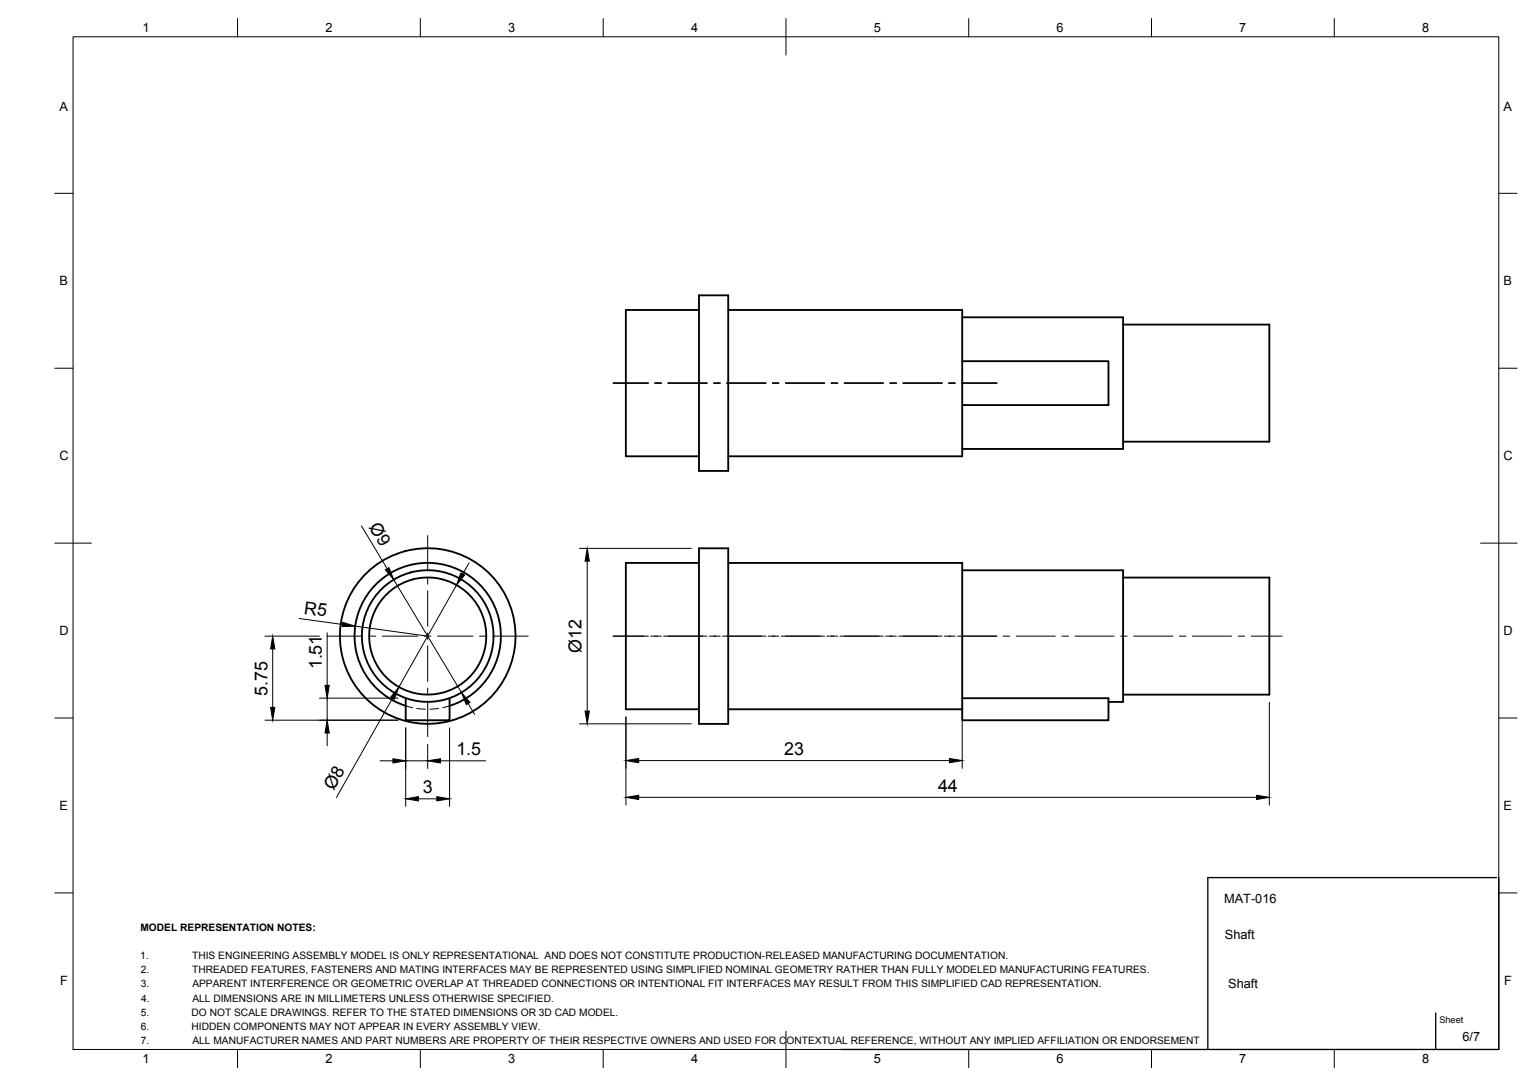
ISO-10303-21;
HEADER;
/* Generated by software containing ST-Developer
 * from STEP Tools, Inc. (www.steptools.com) 
 */

FILE_DESCRIPTION(
/* description */ ('STEP AP214'),
/* implementation_level */ '2;1');

FILE_NAME(
/* name */ 'Shaft.step',
/* time_stamp */ '2026-11-14T06:10:26-08:00',
/* author */ (''),
/* organization */ (''),
/* preprocessor_version */ 'ST-DEVELOPER v20.2',
/* originating_system */ 'Autodesk Translation Framework v15.17.0.0',
/* authorisation */ '');

FILE_SCHEMA (('AUTOMOTIVE_DESIGN { 1 0 10303 214 3 1 1 }'));
ENDSEC;

DATA;
#10=MECHANICAL_DESIGN_GEOMETRIC_PRESENTATION_REPRESENTATION('',(#165),#10413);
#149=SHAPE_REPRESENTATION_RELATIONSHIP('SRR','None',#10454,#157);
#157=ADVANCED_BREP_SHAPE_REPRESENTATION('',(#173),#10406);
#165=STYLED_ITEM('',(#10502),#173);
#173=MANIFOLD_SOLID_BREP('Body1',#5300);
#196=FACE_BOUND('',#606,.T.);
#197=FACE_BOUND('',#608,.T.);
#198=FACE_BOUND('',#611,.T.);
#229=PLANE('',#5455);
#230=PLANE('',#5456);
#231=PLANE('',#5457);
#232=PLANE('',#5458);
#233=PLANE('',#5459);
#234=PLANE('',#5460);
#235=PLANE('',#5461);
#236=PLANE('',#5462);
#237=PLANE('',#5463);
#238=PLANE('',#5464);
#239=PLANE('',#5465);
#294=FACE_OUTER_BOUND('',#600,.T.);
#295=FACE_OUTER_BOUND('',#601,.T.);
#296=FACE_OUTER_BOUND('',#602,.T.);
#297=FACE_OUTER_BOUND('',#603,.T.);
#298=FACE_OUTER_BOUND('',#604,.T.);
#299=FACE_OUTER_BOUND('',#605,.T.);
#300=FACE_OUTER_BOUND('',#607,.T.);
#301=FACE_OUTER_BOUND('',#609,.T.);
#302=FACE_OUTER_BOUND('',#610,.T.);
#303=FACE_OUTER_BOUND('',#612,.T.);
#304=FACE_OUTER_BOUND('',#613,.T.);
#305=FACE_OUTER_BOUND('',#614,.T.);
#306=FACE_OUTER_BOUND('',#615,.T.);
#307=FACE_OUTER_BOUND('',#616,.T.);
#308=FACE_OUTER_BOUND('',#617,.T.);
#309=FACE_OUTER_BOUND('',#618,.T.);
#600=EDGE_LOOP('',(#3312,#3313,#3314,#3315));
#601=EDGE_LOOP('',(#3316,#3317,#3318,#3319,#3320,#3321,#3322,#3323));
#602=EDGE_LOOP('',(#3324,#3325,#3326,#3327,#3328,#3329));
#603=EDGE_LOOP('',(#3330,#3331,#3332,#3333));
#604=EDGE_LOOP('',(#3334,#3335,#3336,#3337));
#605=EDGE_LOOP('',(#3338));
#606=EDGE_LOOP('',(#3339));
#607=EDGE_LOOP('',(#3340));
#608=EDGE_LOOP('',(#3341));
#609=EDGE_LOOP('',(#3342));
#610=EDGE_LOOP('',(#3343));
#611=EDGE_LOOP('',(#3344));
#612=EDGE_LOOP('',(#3345,#3346,#3347,#3348,#3349,#3350));
#613=EDGE_LOOP('',(#3351,#3352,#3353,#3354));
#614=EDGE_LOOP('',(#3355,#3356,#3357,#3358,#3359));
#615=EDGE_LOOP('',(#3360,#3361,#3362,#3363));
#616=EDGE_LOOP('',(#3364,#3365,#3366,#3367,#3368));
#617=EDGE_LOOP('',(#3369,#3370,#3371,#3372));
#618=EDGE_LOOP('',(#3373));
#921=LINE('',#8050,#1212);
#922=LINE('',#8057,#1213);
#923=LINE('',#8061,#1214);
#924=LINE('',#8065,#1215);
#925=LINE('',#8070,#1216);
#926=LINE('',#8080,#1217);
#927=LINE('',#8086,#1218);
#928=LINE('',#8093,#1219);
#929=LINE('',#8094,#1220);
#930=LINE('',#8097,#1221);
#931=LINE('',#8099,#1222);
#932=LINE('',#8100,#1223);
#933=LINE('',#8103,#1224);
#934=LINE('',#8104,#1225);
#935=LINE('',#8107,#1226);
#936=LINE('',#8108,#1227);
#937=LINE('',#8110,#1228);
#1212=VECTOR('',#6261,4.);
#1213=VECTOR('',#6268,1000.);
#1214=VECTOR('',#6271,4.5);
#1215=VECTOR('',#6276,1000.);
#1216=VECTOR('',#6281,5.);
#1217=VECTOR('',#6292,6.);
#1218=VECTOR('',#6299,5.);
#1219=VECTOR('',#6312,1000.);
#1220=VECTOR('',#6313,1000.);
#1221=VECTOR('',#6316,1000.);
#1222=VECTOR('',#6317,1000.);
#1223=VECTOR('',#6318,1000.);
#1224=VECTOR('',#6321,1000.);
#1225=VECTOR('',#6322,1000.);
#1226=VECTOR('',#6325,1000.);
#1227=VECTOR('',#6326,1000.);
#1228=VECTOR('',#6329,1000.);
#1494=CIRCLE('',#5437,4.);
#1495=CIRCLE('',#5438,4.);
#1496=CIRCLE('',#5440,4.5);
#1497=CIRCLE('',#5441,4.5);
#1498=CIRCLE('',#5442,4.5);
#1499=CIRCLE('',#5443,4.5);
#1500=CIRCLE('',#5445,5.);
#1501=CIRCLE('',#5446,5.);
#1502=CIRCLE('',#5447,5.);
#1503=CIRCLE('',#5448,5.);
#1504=CIRCLE('',#5450,6.);
#1505=CIRCLE('',#5451,6.);
#1506=CIRCLE('',#5453,5.);
#1507=CIRCLE('',#5454,5.);
#1947=VERTEX_POINT('',#8047);
#1948=VERTEX_POINT('',#8049);
#1949=VERTEX_POINT('',#8053);
#1950=VERTEX_POINT('',#8054);
#1951=VERTEX_POINT('',#8056);
#1952=VERTEX_POINT('',#8058);
#1953=VERTEX_POINT('',#8060);
#1954=VERTEX_POINT('',#8063);
#1955=VERTEX_POINT('',#8067);
#1956=VERTEX_POINT('',#8069);
#1957=VERTEX_POINT('',#8071);
#1958=VERTEX_POINT('',#8073);
#1959=VERTEX_POINT('',#8077);
#1960=VERTEX_POINT('',#8079);
#1961=VERTEX_POINT('',#8083);
#1962=VERTEX_POINT('',#8085);
#1963=VERTEX_POINT('',#8096);
#1964=VERTEX_POINT('',#8098);
#1965=VERTEX_POINT('',#8102);
#1966=VERTEX_POINT('',#8106);
#2481=EDGE_CURVE('',#1947,#1947,#1494,.T.);
#2482=EDGE_CURVE('',#1947,#1948,#921,.T.);
#2483=EDGE_CURVE('',#1948,#1948,#1495,.T.);
#2484=EDGE_CURVE('',#1949,#1950,#1496,.T.);
#2485=EDGE_CURVE('',#1950,#1951,#922,.T.);
#2486=EDGE_CURVE('',#1951,#1952,#1497,.T.);
#2487=EDGE_CURVE('',#1952,#1953,#923,.T.);
#2488=EDGE_CURVE('',#1953,#1953,#1498,.T.);
#2489=EDGE_CURVE('',#1952,#1954,#1499,.T.);
#2490=EDGE_CURVE('',#1949,#1954,#924,.T.);
#2491=EDGE_CURVE('',#1955,#1955,#1500,.T.);
#2492=EDGE_CURVE('',#1955,#1956,#925,.T.);
#2493=EDGE_CURVE('',#1957,#1956,#1501,.T.);
#2494=EDGE_CURVE('',#1958,#1957,#1502,.T.);
#2495=EDGE_CURVE('',#1956,#1958,#1503,.T.);
#2496=EDGE_CURVE('',#1959,#1959,#1504,.T.);
#2497=EDGE_CURVE('',#1959,#1960,#926,.T.);
#2498=EDGE_CURVE('',#1960,#1960,#1505,.T.);
#2499=EDGE_CURVE('',#1961,#1961,#1506,.T.);
#2500=EDGE_CURVE('',#1961,#1962,#927,.T.);
#2501=EDGE_CURVE('',#1962,#1962,#1507,.T.);
#2502=EDGE_CURVE('',#1954,#1958,#928,.T.);
#2503=EDGE_CURVE('',#1957,#1951,#929,.T.);
#2504=EDGE_CURVE('',#1958,#1963,#930,.T.);
#2505=EDGE_CURVE('',#1964,#1957,#931,.T.);
#2506=EDGE_CURVE('',#1963,#1964,#932,.T.);
#2507=EDGE_CURVE('',#1965,#1963,#933,.T.);
#2508=EDGE_CURVE('',#1949,#1965,#934,.T.);
#2509=EDGE_CURVE('',#1966,#1964,#935,.T.);
#2510=EDGE_CURVE('',#1965,#1966,#936,.T.);
#2511=EDGE_CURVE('',#1966,#1950,#937,.T.);
#3312=ORIENTED_EDGE('',*,*,#2481,.T.);
#3313=ORIENTED_EDGE('',*,*,#2482,.T.);
#3314=ORIENTED_EDGE('',*,*,#2483,.F.);
#3315=ORIENTED_EDGE('',*,*,#2482,.F.);
#3316=ORIENTED_EDGE('',*,*,#2484,.T.);
#3317=ORIENTED_EDGE('',*,*,#2485,.T.);
#3318=ORIENTED_EDGE('',*,*,#2486,.T.);
#3319=ORIENTED_EDGE('',*,*,#2487,.T.);
#3320=ORIENTED_EDGE('',*,*,#2488,.F.);
#3321=ORIENTED_EDGE('',*,*,#2487,.F.);
#3322=ORIENTED_EDGE('',*,*,#2489,.T.);
#3323=ORIENTED_EDGE('',*,*,#2490,.F.);
#3324=ORIENTED_EDGE('',*,*,#2491,.T.);
#3325=ORIENTED_EDGE('',*,*,#2492,.T.);
#3326=ORIENTED_EDGE('',*,*,#2493,.F.);
#3327=ORIENTED_EDGE('',*,*,#2494,.F.);
#3328=ORIENTED_EDGE('',*,*,#2495,.F.);
#3329=ORIENTED_EDGE('',*,*,#2492,.F.);
#3330=ORIENTED_EDGE('',*,*,#2496,.T.);
#3331=ORIENTED_EDGE('',*,*,#2497,.T.);
#3332=ORIENTED_EDGE('',*,*,#2498,.F.);
#3333=ORIENTED_EDGE('',*,*,#2497,.F.);
#3334=ORIENTED_EDGE('',*,*,#2499,.T.);
#3335=ORIENTED_EDGE('',*,*,#2500,.T.);
#3336=ORIENTED_EDGE('',*,*,#2501,.F.);
#3337=ORIENTED_EDGE('',*,*,#2500,.F.);
#3338=ORIENTED_EDGE('',*,*,#2488,.T.);
#3339=ORIENTED_EDGE('',*,*,#2481,.F.);
#3340=ORIENTED_EDGE('',*,*,#2498,.T.);
#3341=ORIENTED_EDGE('',*,*,#2491,.F.);
#3342=ORIENTED_EDGE('',*,*,#2499,.F.);
#3343=ORIENTED_EDGE('',*,*,#2496,.F.);
#3344=ORIENTED_EDGE('',*,*,#2501,.T.);
#3345=ORIENTED_EDGE('',*,*,#2502,.F.);
#3346=ORIENTED_EDGE('',*,*,#2489,.F.);
#3347=ORIENTED_EDGE('',*,*,#2486,.F.);
#3348=ORIENTED_EDGE('',*,*,#2503,.F.);
#3349=ORIENTED_EDGE('',*,*,#2493,.T.);
#3350=ORIENTED_EDGE('',*,*,#2495,.T.);
#3351=ORIENTED_EDGE('',*,*,#2504,.F.);
#3352=ORIENTED_EDGE('',*,*,#2494,.T.);
#3353=ORIENTED_EDGE('',*,*,#2505,.F.);
#3354=ORIENTED_EDGE('',*,*,#2506,.F.);
#3355=ORIENTED_EDGE('',*,*,#2502,.T.);
#3356=ORIENTED_EDGE('',*,*,#2504,.T.);
#3357=ORIENTED_EDGE('',*,*,#2507,.F.);
#3358=ORIENTED_EDGE('',*,*,#2508,.F.);
#3359=ORIENTED_EDGE('',*,*,#2490,.T.);
#3360=ORIENTED_EDGE('',*,*,#2506,.T.);
#3361=ORIENTED_EDGE('',*,*,#2509,.F.);
#3362=ORIENTED_EDGE('',*,*,#2510,.F.);
#3363=ORIENTED_EDGE('',*,*,#2507,.T.);
#3364=ORIENTED_EDGE('',*,*,#2505,.T.);
#3365=ORIENTED_EDGE('',*,*,#2503,.T.);
#3366=ORIENTED_EDGE('',*,*,#2485,.F.);
#3367=ORIENTED_EDGE('',*,*,#2511,.F.);
#3368=ORIENTED_EDGE('',*,*,#2509,.T.);
#3369=ORIENTED_EDGE('',*,*,#2484,.F.);
#3370=ORIENTED_EDGE('',*,*,#2508,.T.);
#3371=ORIENTED_EDGE('',*,*,#2510,.T.);
#3372=ORIENTED_EDGE('',*,*,#2511,.T.);
#3373=ORIENTED_EDGE('',*,*,#2483,.T.);
#4803=CYLINDRICAL_SURFACE('',#5436,4.);
#4804=CYLINDRICAL_SURFACE('',#5439,4.5);
#4805=CYLINDRICAL_SURFACE('',#5444,5.);
#4806=CYLINDRICAL_SURFACE('',#5449,6.);
#4807=CYLINDRICAL_SURFACE('',#5452,5.);
#5028=ADVANCED_FACE('',(#294),#4803,.T.);
#5029=ADVANCED_FACE('',(#295),#4804,.T.);
#5030=ADVANCED_FACE('',(#296),#4805,.T.);
#5031=ADVANCED_FACE('',(#297),#4806,.T.);
#5032=ADVANCED_FACE('',(#298),#4807,.T.);
#5033=ADVANCED_FACE('',(#299,#196),#229,.T.);
#5034=ADVANCED_FACE('',(#300,#197),#230,.T.);
#5035=ADVANCED_FACE('',(#301),#231,.F.);
#5036=ADVANCED_FACE('',(#302,#198),#232,.F.);
#5037=ADVANCED_FACE('',(#303),#233,.T.);
#5038=ADVANCED_FACE('',(#304),#234,.F.);
#5039=ADVANCED_FACE('',(#305),#235,.F.);
#5040=ADVANCED_FACE('',(#306),#236,.F.);
#5041=ADVANCED_FACE('',(#307),#237,.F.);
#5042=ADVANCED_FACE('',(#308),#238,.T.);
#5043=ADVANCED_FACE('',(#309),#239,.T.);
#5300=CLOSED_SHELL('',(#5028,#5029,#5030,#5031,#5032,#5033,#5034,#5035,
#5036,#5037,#5038,#5039,#5040,#5041,#5042,#5043));
#5435=AXIS2_PLACEMENT_3D('',#8045,#6255,#6256);
#5436=AXIS2_PLACEMENT_3D('',#8046,#6257,#6258);
#5437=AXIS2_PLACEMENT_3D('',#8048,#6259,#6260);
#5438=AXIS2_PLACEMENT_3D('',#8051,#6262,#6263);
#5439=AXIS2_PLACEMENT_3D('',#8052,#6264,#6265);
#5440=AXIS2_PLACEMENT_3D('',#8055,#6266,#6267);
#5441=AXIS2_PLACEMENT_3D('',#8059,#6269,#6270);
#5442=AXIS2_PLACEMENT_3D('',#8062,#6272,#6273);
#5443=AXIS2_PLACEMENT_3D('',#8064,#6274,#6275);
#5444=AXIS2_PLACEMENT_3D('',#8066,#6277,#6278);
#5445=AXIS2_PLACEMENT_3D('',#8068,#6279,#6280);
#5446=AXIS2_PLACEMENT_3D('',#8072,#6282,#6283);
#5447=AXIS2_PLACEMENT_3D('',#8074,#6284,#6285);
#5448=AXIS2_PLACEMENT_3D('',#8075,#6286,#6287);
#5449=AXIS2_PLACEMENT_3D('',#8076,#6288,#6289);
#5450=AXIS2_PLACEMENT_3D('',#8078,#6290,#6291);
#5451=AXIS2_PLACEMENT_3D('',#8081,#6293,#6294);
#5452=AXIS2_PLACEMENT_3D('',#8082,#6295,#6296);
#5453=AXIS2_PLACEMENT_3D('',#8084,#6297,#6298);
#5454=AXIS2_PLACEMENT_3D('',#8087,#6300,#6301);
#5455=AXIS2_PLACEMENT_3D('',#8088,#6302,#6303);
#5456=AXIS2_PLACEMENT_3D('',#8089,#6304,#6305);
#5457=AXIS2_PLACEMENT_3D('',#8090,#6306,#6307);
#5458=AXIS2_PLACEMENT_3D('',#8091,#6308,#6309);
#5459=AXIS2_PLACEMENT_3D('',#8092,#6310,#6311);
#5460=AXIS2_PLACEMENT_3D('',#8095,#6314,#6315);
#5461=AXIS2_PLACEMENT_3D('',#8101,#6319,#6320);
#5462=AXIS2_PLACEMENT_3D('',#8105,#6323,#6324);
#5463=AXIS2_PLACEMENT_3D('',#8109,#6327,#6328);
#5464=AXIS2_PLACEMENT_3D('',#8111,#6330,#6331);
#5465=AXIS2_PLACEMENT_3D('',#8112,#6332,#6333);
#6255=DIRECTION('axis',(0.,0.,1.));
#6256=DIRECTION('refdir',(1.,0.,0.));
#6257=DIRECTION('center_axis',(0.,0.,-1.));
#6258=DIRECTION('ref_axis',(-1.,0.,0.));
#6259=DIRECTION('center_axis',(0.,0.,1.));
#6260=DIRECTION('ref_axis',(1.,0.,0.));
#6261=DIRECTION('',(0.,0.,1.));
#6262=DIRECTION('center_axis',(0.,0.,1.));
#6263=DIRECTION('ref_axis',(1.,0.,0.));
#6264=DIRECTION('center_axis',(0.,0.,-1.));
#6265=DIRECTION('ref_axis',(-1.,0.,0.));
#6266=DIRECTION('center_axis',(0.,0.,1.));
#6267=DIRECTION('ref_axis',(1.,0.,0.));
#6268=DIRECTION('',(0.,0.,-1.));
#6269=DIRECTION('center_axis',(0.,0.,1.));
#6270=DIRECTION('ref_axis',(1.,0.,0.));
#6271=DIRECTION('',(0.,0.,1.));
#6272=DIRECTION('center_axis',(0.,0.,1.));
#6273=DIRECTION('ref_axis',(1.,0.,0.));
#6274=DIRECTION('center_axis',(0.,0.,1.));
#6275=DIRECTION('ref_axis',(1.,0.,0.));
#6276=DIRECTION('',(0.,0.,-1.));
#6277=DIRECTION('center_axis',(0.,0.,-1.));
#6278=DIRECTION('ref_axis',(-1.,0.,0.));
#6279=DIRECTION('center_axis',(0.,0.,1.));
#6280=DIRECTION('ref_axis',(1.,0.,0.));
#6281=DIRECTION('',(0.,0.,1.));
#6282=DIRECTION('center_axis',(0.,0.,1.));
#6283=DIRECTION('ref_axis',(1.,0.,0.));
#6284=DIRECTION('center_axis',(0.,0.,1.));
#6285=DIRECTION('ref_axis',(1.,0.,0.));
#6286=DIRECTION('center_axis',(0.,0.,1.));
#6287=DIRECTION('ref_axis',(1.,0.,0.));
#6288=DIRECTION('center_axis',(0.,0.,-1.));
#6289=DIRECTION('ref_axis',(-1.,0.,0.));
#6290=DIRECTION('center_axis',(0.,0.,1.));
#6291=DIRECTION('ref_axis',(1.,0.,0.));
#6292=DIRECTION('',(0.,0.,1.));
#6293=DIRECTION('center_axis',(0.,0.,1.));
#6294=DIRECTION('ref_axis',(1.,0.,0.));
#6295=DIRECTION('center_axis',(0.,0.,-1.));
#6296=DIRECTION('ref_axis',(-1.,0.,0.));
#6297=DIRECTION('center_axis',(0.,0.,1.));
#6298=DIRECTION('ref_axis',(1.,0.,0.));
#6299=DIRECTION('',(0.,0.,1.));
#6300=DIRECTION('center_axis',(0.,0.,1.));
#6301=DIRECTION('ref_axis',(1.,0.,0.));
#6302=DIRECTION('center_axis',(0.,0.,1.));
#6303=DIRECTION('ref_axis',(1.,0.,0.));
#6304=DIRECTION('center_axis',(0.,0.,1.));
#6305=DIRECTION('ref_axis',(1.,0.,0.));
#6306=DIRECTION('center_axis',(0.,0.,1.));
#6307=DIRECTION('ref_axis',(1.,0.,0.));
#6308=DIRECTION('center_axis',(0.,0.,1.));
#6309=DIRECTION('ref_axis',(1.,0.,0.));
#6310=DIRECTION('center_axis',(0.,0.,1.));
#6311=DIRECTION('ref_axis',(1.,0.,0.));
#6312=DIRECTION('',(-1.,0.,0.));
#6313=DIRECTION('',(1.,0.,0.));
#6314=DIRECTION('center_axis',(0.,0.,1.));
#6315=DIRECTION('ref_axis',(1.,0.,0.));
#6316=DIRECTION('',(-1.,0.,0.));
#6317=DIRECTION('',(1.,0.,0.));
#6318=DIRECTION('',(0.,-1.,0.));
#6319=DIRECTION('center_axis',(0.,-1.,0.));
#6320=DIRECTION('ref_axis',(0.,0.,-1.));
#6321=DIRECTION('',(0.,0.,-1.));
#6322=DIRECTION('',(-1.,0.,0.));
#6323=DIRECTION('center_axis',(1.,0.,0.));
#6324=DIRECTION('ref_axis',(0.,0.,-1.));
#6325=DIRECTION('',(0.,0.,-1.));
#6326=DIRECTION('',(0.,-1.,0.));
#6327=DIRECTION('center_axis',(0.,1.,0.));
#6328=DIRECTION('ref_axis',(0.,0.,1.));
#6329=DIRECTION('',(1.,0.,0.));
#6330=DIRECTION('center_axis',(0.,0.,1.));
#6331=DIRECTION('ref_axis',(1.,0.,0.));
#6332=DIRECTION('center_axis',(0.,0.,1.));
#6333=DIRECTION('ref_axis',(1.,0.,0.));
#8045=CARTESIAN_POINT('',(0.,0.,0.));
#8046=CARTESIAN_POINT('Origin',(0.,0.,44.));
#8047=CARTESIAN_POINT('',(4.,-4.89858719658941E-16,34.));
#8048=CARTESIAN_POINT('Origin',(0.,0.,34.));
#8049=CARTESIAN_POINT('',(4.,-4.89858719658941E-16,44.));
#8050=CARTESIAN_POINT('',(4.,-4.89858719658941E-16,44.));
#8051=CARTESIAN_POINT('Origin',(0.,0.,44.));
#8052=CARTESIAN_POINT('Origin',(0.,0.,33.));
#8053=CARTESIAN_POINT('',(-4.24264068711928,1.5,33.));
#8054=CARTESIAN_POINT('',(-4.24264068711928,-1.5,33.));
#8055=CARTESIAN_POINT('Origin',(0.,0.,33.));
#8056=CARTESIAN_POINT('',(-4.24264068711928,-1.5,23.));
#8057=CARTESIAN_POINT('',(-4.24264068711928,-1.5,33.));
#8058=CARTESIAN_POINT('',(4.5,-5.51091059616309E-16,23.));
#8059=CARTESIAN_POINT('Origin',(0.,0.,23.));
#8060=CARTESIAN_POINT('',(4.5,-5.51091059616309E-16,34.));
#8061=CARTESIAN_POINT('',(4.5,-5.51091059616309E-16,33.));
#8062=CARTESIAN_POINT('Origin',(0.,0.,34.));
#8063=CARTESIAN_POINT('',(-4.24264068711929,1.5,23.));
#8064=CARTESIAN_POINT('Origin',(0.,0.,23.));
#8065=CARTESIAN_POINT('',(-4.24264068711929,1.5,33.));
#8066=CARTESIAN_POINT('Origin',(0.,0.,23.));
#8067=CARTESIAN_POINT('',(5.,-6.12323399573677E-16,7.));
#8068=CARTESIAN_POINT('Origin',(0.,0.,7.));
#8069=CARTESIAN_POINT('',(5.,-6.12323399573677E-16,23.));
#8070=CARTESIAN_POINT('',(5.,-6.12323399573677E-16,23.));
#8071=CARTESIAN_POINT('',(-4.76969600708473,-1.5,23.));
#8072=CARTESIAN_POINT('Origin',(0.,0.,23.));
#8073=CARTESIAN_POINT('',(-4.76969600708473,1.5,23.));
#8074=CARTESIAN_POINT('Origin',(0.,0.,23.));
#8075=CARTESIAN_POINT('Origin',(0.,0.,23.));
#8076=CARTESIAN_POINT('Origin',(0.,0.,7.));
#8077=CARTESIAN_POINT('',(6.,-7.34788079488412E-16,5.));
#8078=CARTESIAN_POINT('Origin',(0.,0.,5.));
#8079=CARTESIAN_POINT('',(6.,-7.34788079488412E-16,7.));
#8080=CARTESIAN_POINT('',(6.,-7.34788079488412E-16,7.));
#8081=CARTESIAN_POINT('Origin',(0.,0.,7.));
#8082=CARTESIAN_POINT('Origin',(0.,0.,5.));
#8083=CARTESIAN_POINT('',(5.,-6.12323399573677E-16,0.));
#8084=CARTESIAN_POINT('Origin',(0.,0.,0.));
#8085=CARTESIAN_POINT('',(5.,-6.12323399573677E-16,5.));
#8086=CARTESIAN_POINT('',(5.,-6.12323399573677E-16,5.));
#8087=CARTESIAN_POINT('Origin',(0.,0.,5.));
#8088=CARTESIAN_POINT('Origin',(0.,0.,34.));
#8089=CARTESIAN_POINT('Origin',(0.,0.,7.));
#8090=CARTESIAN_POINT('Origin',(0.,0.,0.));
#8091=CARTESIAN_POINT('Origin',(0.,0.,5.));
#8092=CARTESIAN_POINT('Origin',(0.,0.,23.));
#8093=CARTESIAN_POINT('',(-5.75,1.5,23.));
#8094=CARTESIAN_POINT('',(-5.75,-1.5,23.));
#8095=CARTESIAN_POINT('Origin',(0.,0.,23.));
#8096=CARTESIAN_POINT('',(-5.75,1.5,23.));
#8097=CARTESIAN_POINT('',(-5.75,1.5,23.));
#8098=CARTESIAN_POINT('',(-5.75,-1.5,23.));
#8099=CARTESIAN_POINT('',(-5.75,-1.5,23.));
#8100=CARTESIAN_POINT('',(-5.75,-1.53080849893419E-16,23.));
#8101=CARTESIAN_POINT('Origin',(-5.75,1.5,33.));
#8102=CARTESIAN_POINT('',(-5.75,1.5,33.));
#8103=CARTESIAN_POINT('',(-5.75,1.5,33.));
#8104=CARTESIAN_POINT('',(-5.75,1.5,33.));
#8105=CARTESIAN_POINT('Origin',(-5.75,-1.53080849893419E-16,33.));
#8106=CARTESIAN_POINT('',(-5.75,-1.5,33.));
#8107=CARTESIAN_POINT('',(-5.75,-1.5,33.));
#8108=CARTESIAN_POINT('',(-5.75,-1.53080849893419E-16,33.));
#8109=CARTESIAN_POINT('Origin',(-5.75,-1.5,33.));
#8110=CARTESIAN_POINT('',(-5.75,-1.5,33.));
#8111=CARTESIAN_POINT('Origin',(0.,0.,33.));
#8112=CARTESIAN_POINT('Origin',(0.,0.,44.));
#10396=UNCERTAINTY_MEASURE_WITH_UNIT(LENGTH_MEASURE(0.01),#10414,
'DISTANCE_ACCURACY_VALUE',
'Maximum model space distance between geometric entities at asserted c
onnectivities');
#10403=UNCERTAINTY_MEASURE_WITH_UNIT(LENGTH_MEASURE(0.01),#10414,
'DISTANCE_ACCURACY_VALUE',
'Maximum model space distance between geometric entities at asserted c
onnectivities');
#10406=(
GEOMETRIC_REPRESENTATION_CONTEXT(3)
GLOBAL_UNCERTAINTY_ASSIGNED_CONTEXT((#10396))
GLOBAL_UNIT_ASSIGNED_CONTEXT((#10414,#10416,#10417))
REPRESENTATION_CONTEXT('','3D')
);
#10413=(
GEOMETRIC_REPRESENTATION_CONTEXT(3)
GLOBAL_UNCERTAINTY_ASSIGNED_CONTEXT((#10403))
GLOBAL_UNIT_ASSIGNED_CONTEXT((#10414,#10416,#10417))
REPRESENTATION_CONTEXT('','3D')
);
#10414=(
LENGTH_UNIT()
NAMED_UNIT(*)
SI_UNIT(.MILLI.,.METRE.)
);
#10416=(
NAMED_UNIT(*)
PLANE_ANGLE_UNIT()
SI_UNIT($,.RADIAN.)
);
#10417=(
NAMED_UNIT(*)
SI_UNIT($,.STERADIAN.)
SOLID_ANGLE_UNIT()
);
#10420=SHAPE_DEFINITION_REPRESENTATION(#10429,#10454);
#10429=PRODUCT_DEFINITION_SHAPE('',$,#10464);
#10454=SHAPE_REPRESENTATION('',(#5435),#10406);
#10461=PRODUCT_DEFINITION_CONTEXT('part definition',#10490,'design');
#10464=PRODUCT_DEFINITION('Shaft','Shaft',#10473,#10461);
#10473=PRODUCT_DEFINITION_FORMATION('',$,#10494);
#10490=APPLICATION_CONTEXT(
'Core Data for Automotive Mechanical Design Process');
#10491=PRODUCT_CONTEXT('part definition',#10490,'mechanical');
#10494=PRODUCT('Shaft','Shaft','Shaft',(#10491));
#10502=PRESENTATION_STYLE_ASSIGNMENT((#10506));
#10506=SURFACE_STYLE_USAGE(.BOTH.,#10510);
#10510=SURFACE_SIDE_STYLE('',(#10514));
#10514=SURFACE_STYLE_FILL_AREA(#10518);
#10518=FILL_AREA_STYLE('Opaque(61,176,222)',(#10522));
#10522=FILL_AREA_STYLE_COLOUR('Opaque(61,176,222)',#10526);
#10526=COLOUR_RGB('Opaque(61,176,222)',0.23921568627451,0.690196078431373,
0.870588235294118);
ENDSEC;
END-ISO-10303-21;
